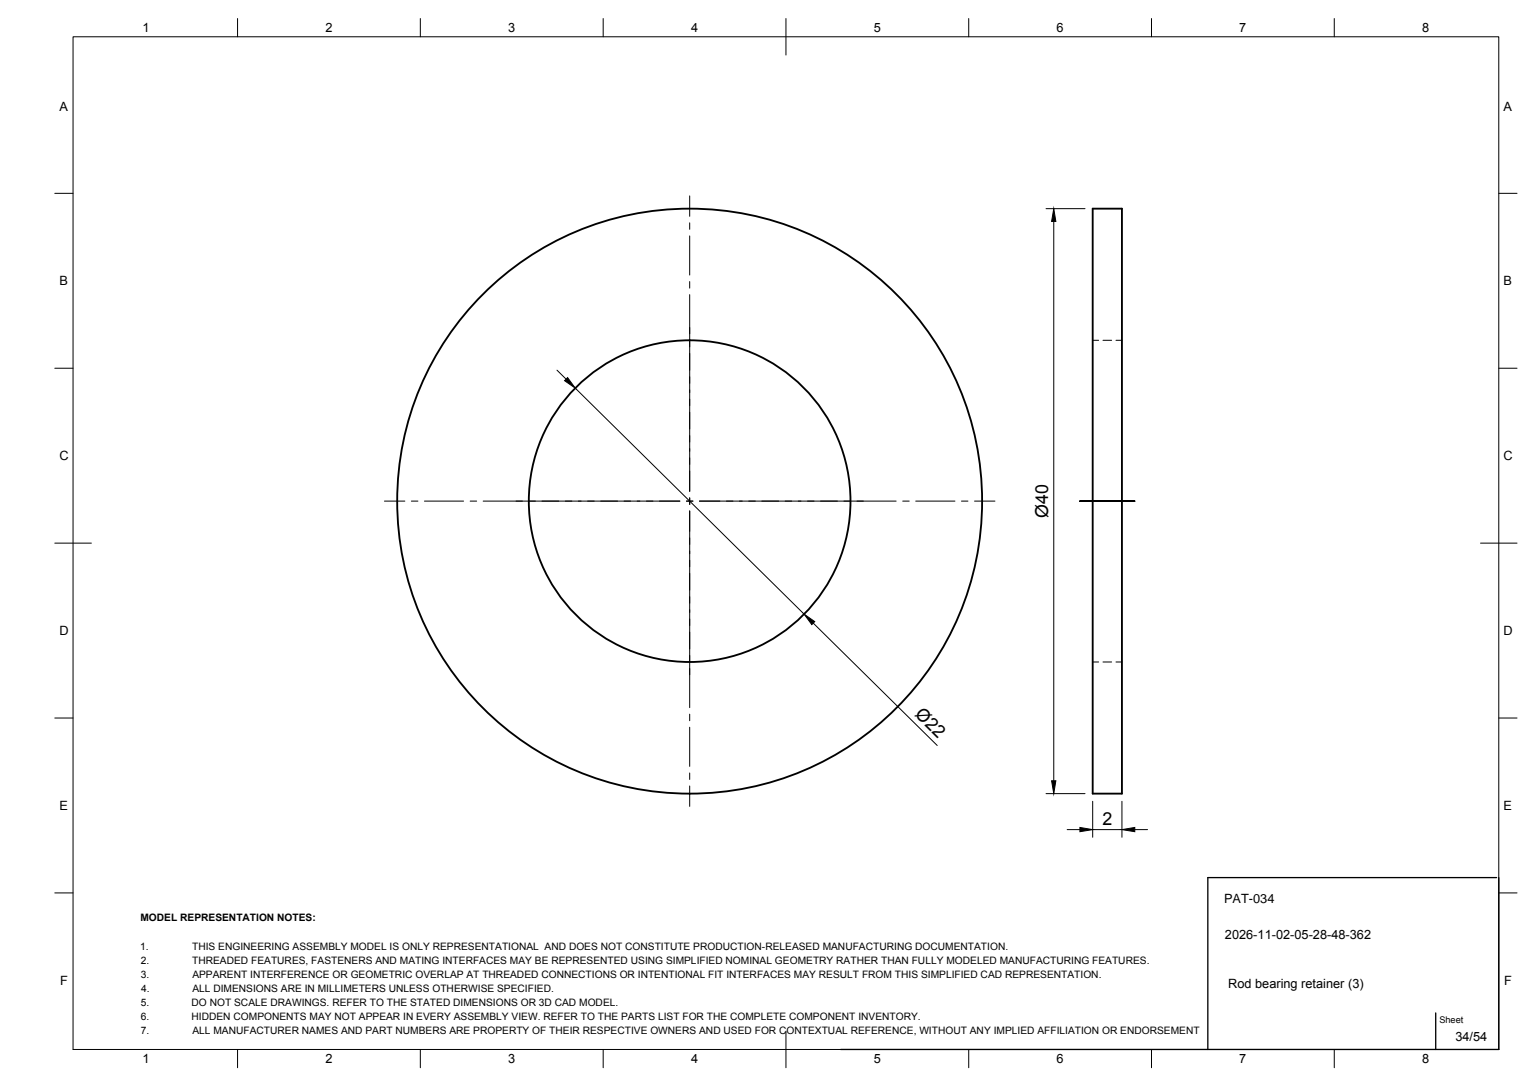
ISO-10303-21;
HEADER;
/* Generated by software containing ST-Developer
 * from STEP Tools, Inc. (www.steptools.com) 
 */

FILE_DESCRIPTION(
/* description */ ('Fatigue rig crank-slider'),
/* implementation_level */ '2;1');

FILE_NAME(
/* name */ 'Rod bearing retainer (3).step',
/* time_stamp */ '2026-10-28T03:24:50-07:00',
/* author */ (''),
/* organization */ (''),
/* preprocessor_version */ 'ST-DEVELOPER v20.2',
/* originating_system */ 'Autodesk Translation Framework v15.17.0.0',
/* authorisation */ '');

FILE_SCHEMA (('AUTOMOTIVE_DESIGN { 1 0 10303 214 3 1 1 }'));
ENDSEC;

DATA;
#10=MECHANICAL_DESIGN_GEOMETRIC_PRESENTATION_REPRESENTATION('',(#619),#16911);
#518=SHAPE_REPRESENTATION_RELATIONSHIP('SRR','None',#17160,#568);
#568=ADVANCED_BREP_SHAPE_REPRESENTATION('',(#676),#16889);
#619=STYLED_ITEM('',(#17487),#676);
#676=MANIFOLD_SOLID_BREP('Body1',#8912);
#852=FACE_BOUND('',#2216,.T.);
#853=FACE_BOUND('',#2218,.T.);
#1092=PLANE('',#10104);
#1093=PLANE('',#10105);
#1538=FACE_OUTER_BOUND('',#2213,.T.);
#1539=FACE_OUTER_BOUND('',#2214,.T.);
#1540=FACE_OUTER_BOUND('',#2215,.T.);
#1541=FACE_OUTER_BOUND('',#2217,.T.);
#2213=EDGE_LOOP('',(#7328,#7329,#7330,#7331));
#2214=EDGE_LOOP('',(#7332,#7333,#7334,#7335));
#2215=EDGE_LOOP('',(#7336));
#2216=EDGE_LOOP('',(#7337));
#2217=EDGE_LOOP('',(#7338));
#2218=EDGE_LOOP('',(#7339));
#2845=LINE('',#15418,#3491);
#2846=LINE('',#15424,#3492);
#3491=VECTOR('',#12165,1.1);
#3492=VECTOR('',#12172,2.);
#3997=CIRCLE('',#10099,1.1);
#3998=CIRCLE('',#10100,1.1);
#3999=CIRCLE('',#10102,2.);
#4000=CIRCLE('',#10103,2.);
#4601=VERTEX_POINT('',#15415);
#4602=VERTEX_POINT('',#15417);
#4603=VERTEX_POINT('',#15421);
#4604=VERTEX_POINT('',#15423);
#5562=EDGE_CURVE('',#4601,#4601,#3997,.T.);
#5563=EDGE_CURVE('',#4601,#4602,#2845,.T.);
#5564=EDGE_CURVE('',#4602,#4602,#3998,.T.);
#5565=EDGE_CURVE('',#4603,#4603,#3999,.T.);
#5566=EDGE_CURVE('',#4603,#4604,#2846,.T.);
#5567=EDGE_CURVE('',#4604,#4604,#4000,.T.);
#7328=ORIENTED_EDGE('',*,*,#5562,.F.);
#7329=ORIENTED_EDGE('',*,*,#5563,.T.);
#7330=ORIENTED_EDGE('',*,*,#5564,.T.);
#7331=ORIENTED_EDGE('',*,*,#5563,.F.);
#7332=ORIENTED_EDGE('',*,*,#5565,.F.);
#7333=ORIENTED_EDGE('',*,*,#5566,.T.);
#7334=ORIENTED_EDGE('',*,*,#5567,.T.);
#7335=ORIENTED_EDGE('',*,*,#5566,.F.);
#7336=ORIENTED_EDGE('',*,*,#5565,.T.);
#7337=ORIENTED_EDGE('',*,*,#5562,.T.);
#7338=ORIENTED_EDGE('',*,*,#5567,.F.);
#7339=ORIENTED_EDGE('',*,*,#5564,.F.);
#8311=CYLINDRICAL_SURFACE('',#10098,1.1);
#8312=CYLINDRICAL_SURFACE('',#10101,2.);
#8676=ADVANCED_FACE('',(#1538),#8311,.F.);
#8677=ADVANCED_FACE('',(#1539),#8312,.T.);
#8678=ADVANCED_FACE('',(#1540,#852),#1092,.T.);
#8679=ADVANCED_FACE('',(#1541,#853),#1093,.F.);
#8912=CLOSED_SHELL('',(#8676,#8677,#8678,#8679));
#10097=AXIS2_PLACEMENT_3D('',#15413,#12159,#12160);
#10098=AXIS2_PLACEMENT_3D('',#15414,#12161,#12162);
#10099=AXIS2_PLACEMENT_3D('',#15416,#12163,#12164);
#10100=AXIS2_PLACEMENT_3D('',#15419,#12166,#12167);
#10101=AXIS2_PLACEMENT_3D('',#15420,#12168,#12169);
#10102=AXIS2_PLACEMENT_3D('',#15422,#12170,#12171);
#10103=AXIS2_PLACEMENT_3D('',#15425,#12173,#12174);
#10104=AXIS2_PLACEMENT_3D('',#15426,#12175,#12176);
#10105=AXIS2_PLACEMENT_3D('',#15427,#12177,#12178);
#12159=DIRECTION('axis',(0.,0.,1.));
#12160=DIRECTION('refdir',(1.,0.,0.));
#12161=DIRECTION('center_axis',(0.,1.,0.));
#12162=DIRECTION('ref_axis',(1.,0.,0.));
#12163=DIRECTION('center_axis',(0.,-1.,0.));
#12164=DIRECTION('ref_axis',(1.,0.,0.));
#12165=DIRECTION('',(0.,-1.,0.));
#12166=DIRECTION('center_axis',(0.,-1.,0.));
#12167=DIRECTION('ref_axis',(1.,0.,0.));
#12168=DIRECTION('center_axis',(0.,1.,0.));
#12169=DIRECTION('ref_axis',(1.,0.,0.));
#12170=DIRECTION('center_axis',(0.,1.,0.));
#12171=DIRECTION('ref_axis',(1.,0.,0.));
#12172=DIRECTION('',(0.,-1.,0.));
#12173=DIRECTION('center_axis',(0.,1.,0.));
#12174=DIRECTION('ref_axis',(1.,0.,0.));
#12175=DIRECTION('center_axis',(0.,1.,0.));
#12176=DIRECTION('ref_axis',(1.,0.,0.));
#12177=DIRECTION('center_axis',(0.,1.,0.));
#12178=DIRECTION('ref_axis',(1.,0.,0.));
#15413=CARTESIAN_POINT('',(0.,0.,0.));
#15414=CARTESIAN_POINT('Origin',(11.,4.4,12.));
#15415=CARTESIAN_POINT('',(9.9,4.6,12.));
#15416=CARTESIAN_POINT('Origin',(11.,4.6,12.));
#15417=CARTESIAN_POINT('',(9.9,4.4,12.));
#15418=CARTESIAN_POINT('',(9.9,4.4,12.));
#15419=CARTESIAN_POINT('Origin',(11.,4.4,12.));
#15420=CARTESIAN_POINT('Origin',(11.,4.4,12.));
#15421=CARTESIAN_POINT('',(9.,4.6,12.));
#15422=CARTESIAN_POINT('Origin',(11.,4.6,12.));
#15423=CARTESIAN_POINT('',(9.,4.4,12.));
#15424=CARTESIAN_POINT('',(9.,4.4,12.));
#15425=CARTESIAN_POINT('Origin',(11.,4.4,12.));
#15426=CARTESIAN_POINT('Origin',(11.,4.6,12.));
#15427=CARTESIAN_POINT('Origin',(11.,4.4,12.));
#16830=UNCERTAINTY_MEASURE_WITH_UNIT(LENGTH_MEASURE(0.001),#16912,
'DISTANCE_ACCURACY_VALUE',
'Maximum model space distance between geometric entities at asserted c
onnectivities');
#16852=UNCERTAINTY_MEASURE_WITH_UNIT(LENGTH_MEASURE(0.001),#16912,
'DISTANCE_ACCURACY_VALUE',
'Maximum model space distance between geometric entities at asserted c
onnectivities');
#16889=(
GEOMETRIC_REPRESENTATION_CONTEXT(3)
GLOBAL_UNCERTAINTY_ASSIGNED_CONTEXT((#16830))
GLOBAL_UNIT_ASSIGNED_CONTEXT((#16912,#16914,#16915))
REPRESENTATION_CONTEXT('','3D')
);
#16911=(
GEOMETRIC_REPRESENTATION_CONTEXT(3)
GLOBAL_UNCERTAINTY_ASSIGNED_CONTEXT((#16852))
GLOBAL_UNIT_ASSIGNED_CONTEXT((#16912,#16914,#16915))
REPRESENTATION_CONTEXT('','3D')
);
#16912=(
LENGTH_UNIT()
NAMED_UNIT(*)
SI_UNIT(.CENTI.,.METRE.)
);
#16914=(
NAMED_UNIT(*)
PLANE_ANGLE_UNIT()
SI_UNIT($,.RADIAN.)
);
#16915=(
NAMED_UNIT(*)
SI_UNIT($,.STERADIAN.)
SOLID_ANGLE_UNIT()
);
#16952=SHAPE_DEFINITION_REPRESENTATION(#17012,#17160);
#17012=PRODUCT_DEFINITION_SHAPE('',$,#17219);
#17160=SHAPE_REPRESENTATION('',(#10097),#16889);
#17182=PRODUCT_DEFINITION_CONTEXT('part definition',#17358,'design');
#17219=PRODUCT_DEFINITION('Rod bearing retainer (3)',
'Rod bearing retainer (3)',#17277,#17182);
#17277=PRODUCT_DEFINITION_FORMATION('',$,#17396);
#17358=APPLICATION_CONTEXT(
'Core Data for Automotive Mechanical Design Process');
#17359=PRODUCT_CONTEXT('part definition',#17358,'mechanical');
#17396=PRODUCT('Rod bearing retainer (3)','Rod bearing retainer (3)',
'Rod bearing retainer (3)',(#17359));
#17481=COLOUR_RGB('Grey',0.48,0.52,0.57);
#17482=FILL_AREA_STYLE_COLOUR('',#17481);
#17483=FILL_AREA_STYLE('',(#17482));
#17484=SURFACE_STYLE_FILL_AREA(#17483);
#17485=SURFACE_SIDE_STYLE('',(#17484));
#17486=SURFACE_STYLE_USAGE(.BOTH.,#17485);
#17487=PRESENTATION_STYLE_ASSIGNMENT((#17486));
ENDSEC;
END-ISO-10303-21;
